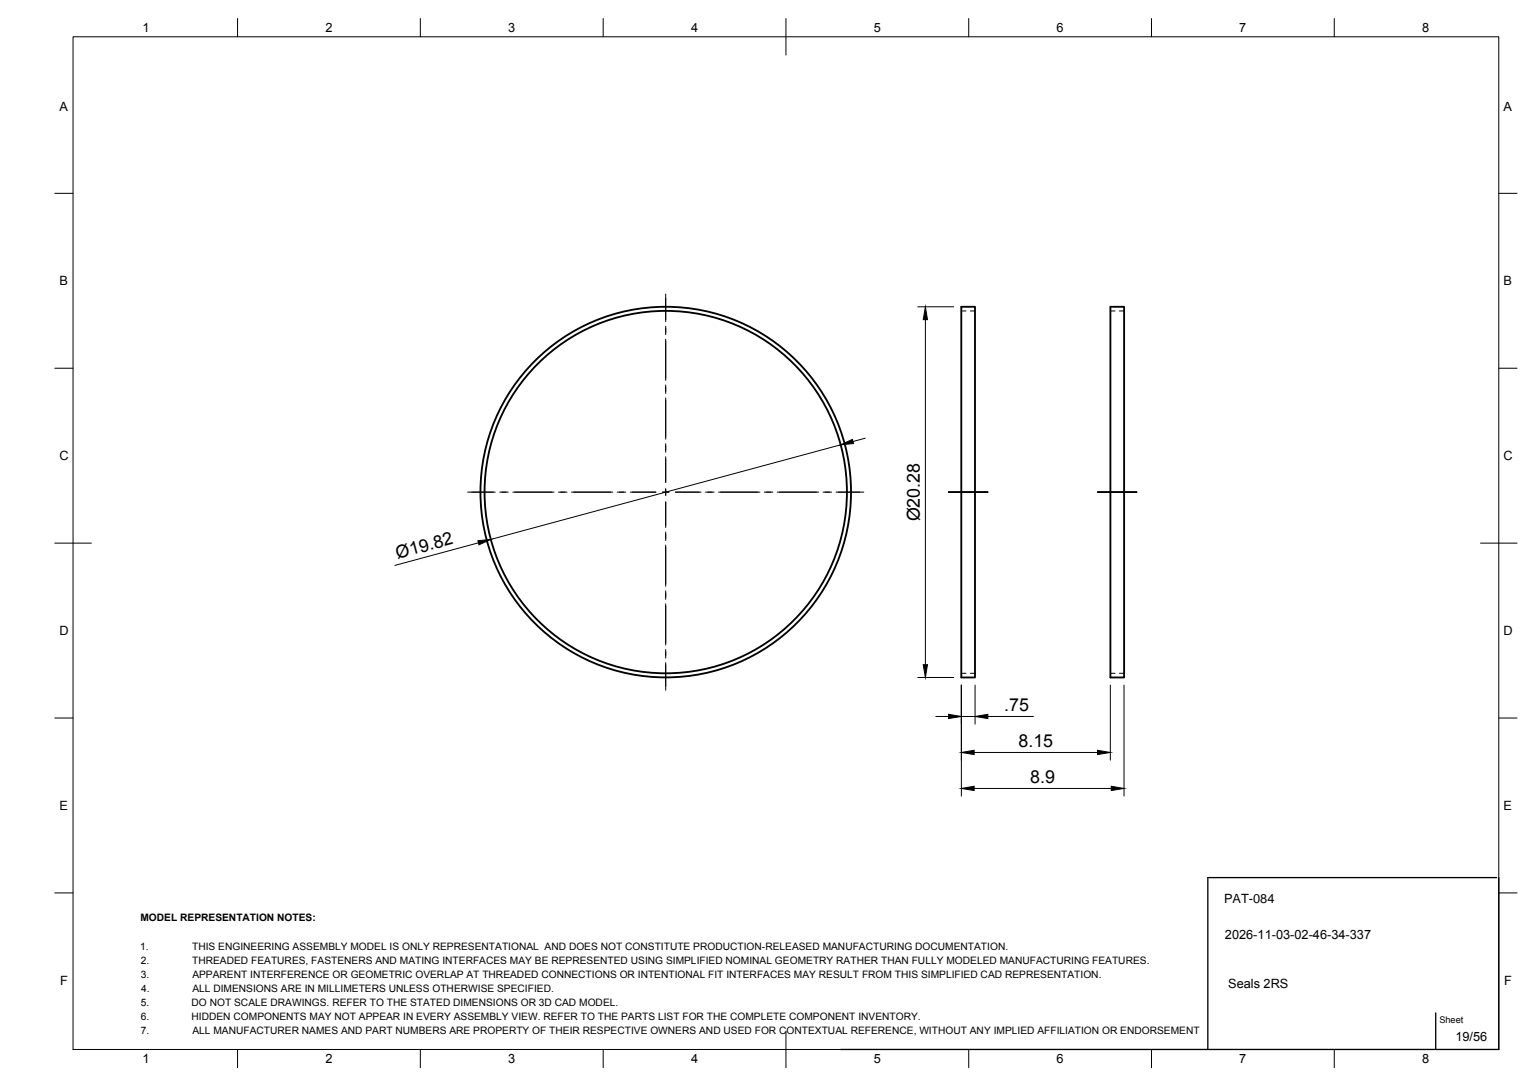
ISO-10303-21;
HEADER;
/* Generated by software containing ST-Developer
 * from STEP Tools, Inc. (www.steptools.com) 
 */

FILE_DESCRIPTION(
/* description */ ('Quick-return (Whitworth) mechanism'),
/* implementation_level */ '2;1');

FILE_NAME(
/* name */ 'Seals 2RS.step',
/* time_stamp */ '2026-10-28T03:25:57-07:00',
/* author */ (''),
/* organization */ (''),
/* preprocessor_version */ 'ST-DEVELOPER v20.2',
/* originating_system */ 'Autodesk Translation Framework v15.17.0.0',
/* authorisation */ '');

FILE_SCHEMA (('AUTOMOTIVE_DESIGN { 1 0 10303 214 3 1 1 }'));
ENDSEC;

DATA;
#10=MECHANICAL_DESIGN_GEOMETRIC_PRESENTATION_REPRESENTATION('',(#509,#510),#14878);
#414=SHAPE_REPRESENTATION_RELATIONSHIP('SRR','None',#15083,#458);
#458=ADVANCED_BREP_SHAPE_REPRESENTATION('',(#561,#562),#14840);
#509=STYLED_ITEM('',(#15406),#561);
#510=STYLED_ITEM('',(#15406),#562);
#561=MANIFOLD_SOLID_BREP('Body1',#7863);
#562=MANIFOLD_SOLID_BREP('Body2',#7864);
#698=FACE_BOUND('',#1814,.T.);
#699=FACE_BOUND('',#1817,.T.);
#700=FACE_BOUND('',#1820,.T.);
#701=FACE_BOUND('',#1823,.T.);
#869=PLANE('',#8821);
#870=PLANE('',#8826);
#871=PLANE('',#8829);
#872=PLANE('',#8834);
#1240=FACE_OUTER_BOUND('',#1813,.T.);
#1241=FACE_OUTER_BOUND('',#1815,.T.);
#1242=FACE_OUTER_BOUND('',#1816,.T.);
#1243=FACE_OUTER_BOUND('',#1818,.T.);
#1244=FACE_OUTER_BOUND('',#1819,.T.);
#1245=FACE_OUTER_BOUND('',#1821,.T.);
#1246=FACE_OUTER_BOUND('',#1822,.T.);
#1247=FACE_OUTER_BOUND('',#1824,.T.);
#1813=EDGE_LOOP('',(#6106));
#1814=EDGE_LOOP('',(#6107));
#1815=EDGE_LOOP('',(#6108,#6109,#6110,#6111));
#1816=EDGE_LOOP('',(#6112));
#1817=EDGE_LOOP('',(#6113));
#1818=EDGE_LOOP('',(#6114,#6115,#6116,#6117));
#1819=EDGE_LOOP('',(#6118));
#1820=EDGE_LOOP('',(#6119));
#1821=EDGE_LOOP('',(#6120,#6121,#6122,#6123));
#1822=EDGE_LOOP('',(#6124));
#1823=EDGE_LOOP('',(#6125));
#1824=EDGE_LOOP('',(#6126,#6127,#6128,#6129));
#2338=LINE('',#13351,#2861);
#2339=LINE('',#13356,#2862);
#2340=LINE('',#13365,#2863);
#2341=LINE('',#13370,#2864);
#2861=VECTOR('',#10449,1.013815);
#2862=VECTOR('',#10456,0.991185);
#2863=VECTOR('',#10467,1.013815);
#2864=VECTOR('',#10474,0.991185);
#3444=CIRCLE('',#8822,1.013815);
#3445=CIRCLE('',#8823,0.991185);
#3446=CIRCLE('',#8825,1.013815);
#3447=CIRCLE('',#8827,0.991185);
#3448=CIRCLE('',#8830,1.013815);
#3449=CIRCLE('',#8831,0.991185);
#3450=CIRCLE('',#8833,1.013815);
#3451=CIRCLE('',#8835,0.991185);
#3923=VERTEX_POINT('',#13344);
#3924=VERTEX_POINT('',#13346);
#3925=VERTEX_POINT('',#13349);
#3926=VERTEX_POINT('',#13353);
#3927=VERTEX_POINT('',#13358);
#3928=VERTEX_POINT('',#13360);
#3929=VERTEX_POINT('',#13363);
#3930=VERTEX_POINT('',#13367);
#4710=EDGE_CURVE('',#3923,#3923,#3444,.T.);
#4711=EDGE_CURVE('',#3924,#3924,#3445,.T.);
#4712=EDGE_CURVE('',#3925,#3925,#3446,.T.);
#4713=EDGE_CURVE('',#3925,#3923,#2338,.T.);
#4714=EDGE_CURVE('',#3926,#3926,#3447,.T.);
#4715=EDGE_CURVE('',#3926,#3924,#2339,.T.);
#4716=EDGE_CURVE('',#3927,#3927,#3448,.T.);
#4717=EDGE_CURVE('',#3928,#3928,#3449,.T.);
#4718=EDGE_CURVE('',#3929,#3929,#3450,.T.);
#4719=EDGE_CURVE('',#3929,#3927,#2340,.T.);
#4720=EDGE_CURVE('',#3930,#3930,#3451,.T.);
#4721=EDGE_CURVE('',#3930,#3928,#2341,.T.);
#6106=ORIENTED_EDGE('',*,*,#4710,.F.);
#6107=ORIENTED_EDGE('',*,*,#4711,.T.);
#6108=ORIENTED_EDGE('',*,*,#4712,.F.);
#6109=ORIENTED_EDGE('',*,*,#4713,.T.);
#6110=ORIENTED_EDGE('',*,*,#4710,.T.);
#6111=ORIENTED_EDGE('',*,*,#4713,.F.);
#6112=ORIENTED_EDGE('',*,*,#4712,.T.);
#6113=ORIENTED_EDGE('',*,*,#4714,.F.);
#6114=ORIENTED_EDGE('',*,*,#4714,.T.);
#6115=ORIENTED_EDGE('',*,*,#4715,.T.);
#6116=ORIENTED_EDGE('',*,*,#4711,.F.);
#6117=ORIENTED_EDGE('',*,*,#4715,.F.);
#6118=ORIENTED_EDGE('',*,*,#4716,.F.);
#6119=ORIENTED_EDGE('',*,*,#4717,.T.);
#6120=ORIENTED_EDGE('',*,*,#4718,.F.);
#6121=ORIENTED_EDGE('',*,*,#4719,.T.);
#6122=ORIENTED_EDGE('',*,*,#4716,.T.);
#6123=ORIENTED_EDGE('',*,*,#4719,.F.);
#6124=ORIENTED_EDGE('',*,*,#4718,.T.);
#6125=ORIENTED_EDGE('',*,*,#4720,.F.);
#6126=ORIENTED_EDGE('',*,*,#4720,.T.);
#6127=ORIENTED_EDGE('',*,*,#4721,.T.);
#6128=ORIENTED_EDGE('',*,*,#4717,.F.);
#6129=ORIENTED_EDGE('',*,*,#4721,.F.);
#7294=CYLINDRICAL_SURFACE('',#8824,1.013815);
#7295=CYLINDRICAL_SURFACE('',#8828,0.991185);
#7296=CYLINDRICAL_SURFACE('',#8832,1.013815);
#7297=CYLINDRICAL_SURFACE('',#8836,0.991185);
#7571=ADVANCED_FACE('',(#1240,#698),#869,.T.);
#7572=ADVANCED_FACE('',(#1241),#7294,.T.);
#7573=ADVANCED_FACE('',(#1242,#699),#870,.T.);
#7574=ADVANCED_FACE('',(#1243),#7295,.F.);
#7575=ADVANCED_FACE('',(#1244,#700),#871,.T.);
#7576=ADVANCED_FACE('',(#1245),#7296,.T.);
#7577=ADVANCED_FACE('',(#1246,#701),#872,.T.);
#7578=ADVANCED_FACE('',(#1247),#7297,.F.);
#7863=CLOSED_SHELL('',(#7571,#7572,#7573,#7574));
#7864=CLOSED_SHELL('',(#7575,#7576,#7577,#7578));
#8820=AXIS2_PLACEMENT_3D('',#13342,#10437,#10438);
#8821=AXIS2_PLACEMENT_3D('',#13343,#10439,#10440);
#8822=AXIS2_PLACEMENT_3D('',#13345,#10441,#10442);
#8823=AXIS2_PLACEMENT_3D('',#13347,#10443,#10444);
#8824=AXIS2_PLACEMENT_3D('',#13348,#10445,#10446);
#8825=AXIS2_PLACEMENT_3D('',#13350,#10447,#10448);
#8826=AXIS2_PLACEMENT_3D('',#13352,#10450,#10451);
#8827=AXIS2_PLACEMENT_3D('',#13354,#10452,#10453);
#8828=AXIS2_PLACEMENT_3D('',#13355,#10454,#10455);
#8829=AXIS2_PLACEMENT_3D('',#13357,#10457,#10458);
#8830=AXIS2_PLACEMENT_3D('',#13359,#10459,#10460);
#8831=AXIS2_PLACEMENT_3D('',#13361,#10461,#10462);
#8832=AXIS2_PLACEMENT_3D('',#13362,#10463,#10464);
#8833=AXIS2_PLACEMENT_3D('',#13364,#10465,#10466);
#8834=AXIS2_PLACEMENT_3D('',#13366,#10468,#10469);
#8835=AXIS2_PLACEMENT_3D('',#13368,#10470,#10471);
#8836=AXIS2_PLACEMENT_3D('',#13369,#10472,#10473);
#10437=DIRECTION('axis',(0.,0.,1.));
#10438=DIRECTION('refdir',(1.,0.,0.));
#10439=DIRECTION('center_axis',(0.,1.,0.));
#10440=DIRECTION('ref_axis',(0.,0.,1.));
#10441=DIRECTION('center_axis',(0.,-1.,0.));
#10442=DIRECTION('ref_axis',(1.,0.,0.));
#10443=DIRECTION('center_axis',(0.,-1.,0.));
#10444=DIRECTION('ref_axis',(1.,0.,0.));
#10445=DIRECTION('center_axis',(0.,-1.,0.));
#10446=DIRECTION('ref_axis',(1.,0.,0.));
#10447=DIRECTION('center_axis',(0.,-1.,0.));
#10448=DIRECTION('ref_axis',(1.,0.,0.));
#10449=DIRECTION('',(0.,1.,0.));
#10450=DIRECTION('center_axis',(0.,-1.,0.));
#10451=DIRECTION('ref_axis',(0.,0.,-1.));
#10452=DIRECTION('center_axis',(0.,-1.,0.));
#10453=DIRECTION('ref_axis',(1.,0.,0.));
#10454=DIRECTION('center_axis',(0.,-1.,0.));
#10455=DIRECTION('ref_axis',(1.,0.,0.));
#10456=DIRECTION('',(0.,1.,0.));
#10457=DIRECTION('center_axis',(0.,1.,0.));
#10458=DIRECTION('ref_axis',(0.,0.,1.));
#10459=DIRECTION('center_axis',(0.,-1.,0.));
#10460=DIRECTION('ref_axis',(1.,0.,0.));
#10461=DIRECTION('center_axis',(0.,-1.,0.));
#10462=DIRECTION('ref_axis',(1.,0.,0.));
#10463=DIRECTION('center_axis',(0.,-1.,0.));
#10464=DIRECTION('ref_axis',(1.,0.,0.));
#10465=DIRECTION('center_axis',(0.,-1.,0.));
#10466=DIRECTION('ref_axis',(1.,0.,0.));
#10467=DIRECTION('',(0.,1.,0.));
#10468=DIRECTION('center_axis',(0.,-1.,0.));
#10469=DIRECTION('ref_axis',(0.,0.,-1.));
#10470=DIRECTION('center_axis',(0.,-1.,0.));
#10471=DIRECTION('ref_axis',(1.,0.,0.));
#10472=DIRECTION('center_axis',(0.,-1.,0.));
#10473=DIRECTION('ref_axis',(1.,0.,0.));
#10474=DIRECTION('',(0.,1.,0.));
#13342=CARTESIAN_POINT('',(0.,0.,0.));
#13343=CARTESIAN_POINT('Origin',(1.013815,0.445,0.));
#13344=CARTESIAN_POINT('',(-1.013815,0.445,-1.24156529467757E-16));
#13345=CARTESIAN_POINT('Origin',(0.,0.445,0.));
#13346=CARTESIAN_POINT('',(-0.991185,0.445,-1.21385153761287E-16));
#13347=CARTESIAN_POINT('Origin',(0.,0.445,0.));
#13348=CARTESIAN_POINT('Origin',(0.,0.4075,0.));
#13349=CARTESIAN_POINT('',(-1.013815,0.37,-1.24156529467757E-16));
#13350=CARTESIAN_POINT('Origin',(0.,0.37,0.));
#13351=CARTESIAN_POINT('',(-1.013815,0.4075,-1.24156529467757E-16));
#13352=CARTESIAN_POINT('Origin',(0.991185,0.37,0.));
#13353=CARTESIAN_POINT('',(-0.991185,0.37,-1.21385153761287E-16));
#13354=CARTESIAN_POINT('Origin',(0.,0.37,0.));
#13355=CARTESIAN_POINT('Origin',(0.,0.4075,0.));
#13356=CARTESIAN_POINT('',(-0.991185,0.4075,-1.21385153761287E-16));
#13357=CARTESIAN_POINT('Origin',(1.013815,-0.37,0.));
#13358=CARTESIAN_POINT('',(-1.013815,-0.37,-1.24156529467757E-16));
#13359=CARTESIAN_POINT('Origin',(0.,-0.37,0.));
#13360=CARTESIAN_POINT('',(-0.991185,-0.37,-1.21385153761287E-16));
#13361=CARTESIAN_POINT('Origin',(0.,-0.37,0.));
#13362=CARTESIAN_POINT('Origin',(0.,-0.4075,0.));
#13363=CARTESIAN_POINT('',(-1.013815,-0.445,-1.24156529467757E-16));
#13364=CARTESIAN_POINT('Origin',(0.,-0.445,0.));
#13365=CARTESIAN_POINT('',(-1.013815,-0.4075,-1.24156529467757E-16));
#13366=CARTESIAN_POINT('Origin',(0.991185,-0.445,0.));
#13367=CARTESIAN_POINT('',(-0.991185,-0.445,-1.21385153761287E-16));
#13368=CARTESIAN_POINT('Origin',(0.,-0.445,0.));
#13369=CARTESIAN_POINT('Origin',(0.,-0.4075,0.));
#13370=CARTESIAN_POINT('',(-0.991185,-0.4075,-1.21385153761287E-16));
#14786=UNCERTAINTY_MEASURE_WITH_UNIT(LENGTH_MEASURE(0.001),#14879,
'DISTANCE_ACCURACY_VALUE',
'Maximum model space distance between geometric entities at asserted c
onnectivities');
#14824=UNCERTAINTY_MEASURE_WITH_UNIT(LENGTH_MEASURE(0.001),#14879,
'DISTANCE_ACCURACY_VALUE',
'Maximum model space distance between geometric entities at asserted c
onnectivities');
#14840=(
GEOMETRIC_REPRESENTATION_CONTEXT(3)
GLOBAL_UNCERTAINTY_ASSIGNED_CONTEXT((#14786))
GLOBAL_UNIT_ASSIGNED_CONTEXT((#14879,#14881,#14882))
REPRESENTATION_CONTEXT('','3D')
);
#14878=(
GEOMETRIC_REPRESENTATION_CONTEXT(3)
GLOBAL_UNCERTAINTY_ASSIGNED_CONTEXT((#14824))
GLOBAL_UNIT_ASSIGNED_CONTEXT((#14879,#14881,#14882))
REPRESENTATION_CONTEXT('','3D')
);
#14879=(
LENGTH_UNIT()
NAMED_UNIT(*)
SI_UNIT(.CENTI.,.METRE.)
);
#14881=(
NAMED_UNIT(*)
PLANE_ANGLE_UNIT()
SI_UNIT($,.RADIAN.)
);
#14882=(
NAMED_UNIT(*)
SI_UNIT($,.STERADIAN.)
SOLID_ANGLE_UNIT()
);
#14898=SHAPE_DEFINITION_REPRESENTATION(#14951,#15083);
#14951=PRODUCT_DEFINITION_SHAPE('',$,#15137);
#15083=SHAPE_REPRESENTATION('',(#8820),#14840);
#15121=PRODUCT_DEFINITION_CONTEXT('part definition',#15282,'design');
#15137=PRODUCT_DEFINITION('Seals 2RS','Seals 2RS',#15190,#15121);
#15190=PRODUCT_DEFINITION_FORMATION('',$,#15299);
#15282=APPLICATION_CONTEXT(
'Core Data for Automotive Mechanical Design Process');
#15283=PRODUCT_CONTEXT('part definition',#15282,'mechanical');
#15299=PRODUCT('Seals 2RS','Seals 2RS','Seals 2RS',(#15283));
#15400=COLOUR_RGB('Grey',0.48,0.52,0.57);
#15401=FILL_AREA_STYLE_COLOUR('',#15400);
#15402=FILL_AREA_STYLE('',(#15401));
#15403=SURFACE_STYLE_FILL_AREA(#15402);
#15404=SURFACE_SIDE_STYLE('',(#15403));
#15405=SURFACE_STYLE_USAGE(.BOTH.,#15404);
#15406=PRESENTATION_STYLE_ASSIGNMENT((#15405));
ENDSEC;
END-ISO-10303-21;
